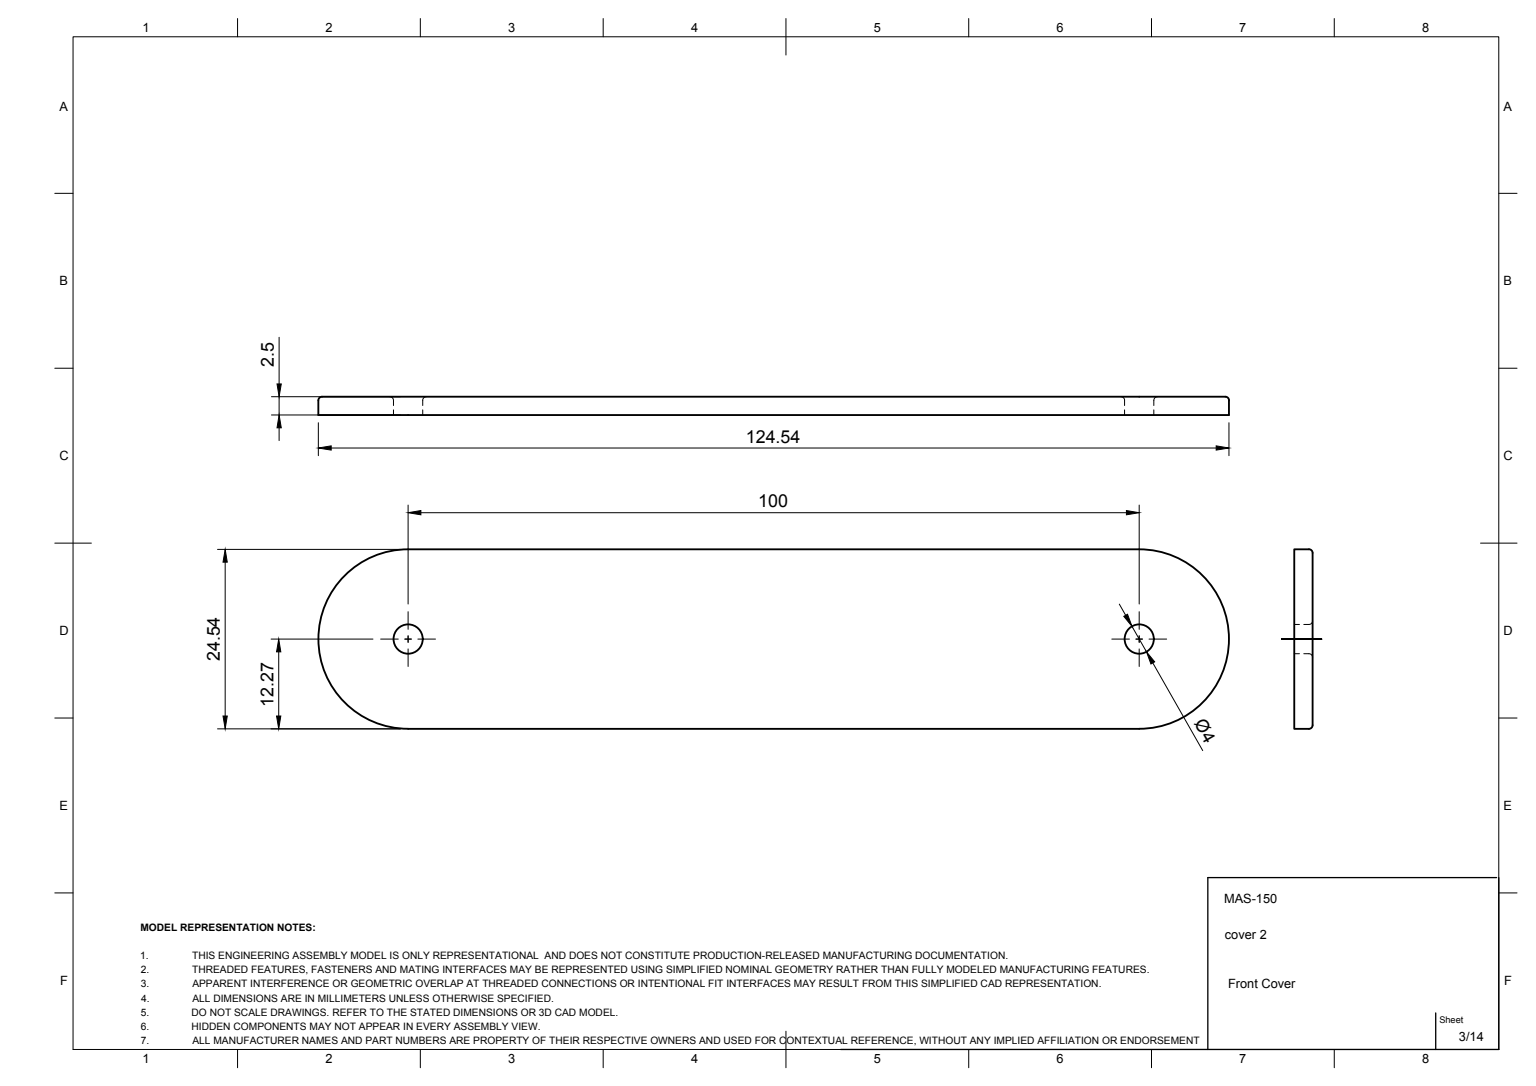
ISO-10303-21;
HEADER;
/* Generated by software containing ST-Developer
 * from STEP Tools, Inc. (www.steptools.com) 
 */

FILE_DESCRIPTION(
/* description */ ('STEP AP203'),
/* implementation_level */ '2;1');

FILE_NAME(
/* name */ 'Front Cover.step',
/* time_stamp */ '2026-11-08T21:40:52-08:00',
/* author */ (''),
/* organization */ (''),
/* preprocessor_version */ 'ST-DEVELOPER v20.2',
/* originating_system */ 'Autodesk Translation Framework v15.17.0.0',
/* authorisation */ '');

FILE_SCHEMA (('AUTOMOTIVE_DESIGN { 1 0 10303 214 3 1 1 }'));
ENDSEC;

DATA;
#10=MECHANICAL_DESIGN_GEOMETRIC_PRESENTATION_REPRESENTATION('',(#183),#12137);
#161=SHAPE_REPRESENTATION_RELATIONSHIP('SRR','None',#12184,#172);
#172=ADVANCED_BREP_SHAPE_REPRESENTATION('',(#194),#12125);
#183=STYLED_ITEM('',(#12253),#194);
#194=MANIFOLD_SOLID_BREP('Body1',#1828);
#205=FACE_BOUND('',#605,.T.);
#206=FACE_BOUND('',#606,.T.);
#207=FACE_BOUND('',#608,.T.);
#208=FACE_BOUND('',#609,.T.);
#232=PLANE('',#1977);
#233=PLANE('',#1980);
#234=PLANE('',#1985);
#235=PLANE('',#1988);
#276=LINE('',#2672,#370);
#277=LINE('',#2676,#371);
#278=LINE('',#2683,#372);
#279=LINE('',#2686,#373);
#280=LINE('',#2692,#374);
#281=LINE('',#2695,#375);
#282=LINE('',#2698,#376);
#283=LINE('',#2701,#377);
#284=LINE('',#2704,#378);
#285=LINE('',#2705,#379);
#286=LINE('',#2708,#380);
#287=LINE('',#2711,#381);
#370=VECTOR('',#2186,2.);
#371=VECTOR('',#2191,2.);
#372=VECTOR('',#2198,1000.);
#373=VECTOR('',#2201,1000.);
#374=VECTOR('',#2206,1000.);
#375=VECTOR('',#2209,1000.);
#376=VECTOR('',#2212,1000.);
#377=VECTOR('',#2215,1000.);
#378=VECTOR('',#2218,1000.);
#379=VECTOR('',#2219,1000.);
#380=VECTOR('',#2222,1000.);
#381=VECTOR('',#2227,1000.);
#464=CYLINDRICAL_SURFACE('',#1973,2.);
#465=CYLINDRICAL_SURFACE('',#1975,2.);
#466=CYLINDRICAL_SURFACE('',#1983,12.2723008899906);
#467=CYLINDRICAL_SURFACE('',#1986,12.2723008899906);
#468=CYLINDRICAL_SURFACE('',#1989,0.5);
#469=CYLINDRICAL_SURFACE('',#1996,0.5);
#490=FACE_OUTER_BOUND('',#600,.T.);
#491=FACE_OUTER_BOUND('',#601,.T.);
#492=FACE_OUTER_BOUND('',#602,.T.);
#493=FACE_OUTER_BOUND('',#603,.T.);
#494=FACE_OUTER_BOUND('',#604,.T.);
#495=FACE_OUTER_BOUND('',#607,.T.);
#496=FACE_OUTER_BOUND('',#610,.T.);
#497=FACE_OUTER_BOUND('',#611,.T.);
#498=FACE_OUTER_BOUND('',#612,.T.);
#499=FACE_OUTER_BOUND('',#613,.T.);
#500=FACE_OUTER_BOUND('',#614,.T.);
#501=FACE_OUTER_BOUND('',#615,.T.);
#502=FACE_OUTER_BOUND('',#616,.T.);
#503=FACE_OUTER_BOUND('',#617,.T.);
#600=EDGE_LOOP('',(#1223,#1224,#1225,#1226,#1227));
#601=EDGE_LOOP('',(#1228,#1229,#1230,#1231,#1232));
#602=EDGE_LOOP('',(#1233,#1234,#1235,#1236,#1237));
#603=EDGE_LOOP('',(#1238,#1239,#1240,#1241,#1242));
#604=EDGE_LOOP('',(#1243,#1244,#1245,#1246));
#605=EDGE_LOOP('',(#1247));
#606=EDGE_LOOP('',(#1248));
#607=EDGE_LOOP('',(#1249,#1250,#1251,#1252));
#608=EDGE_LOOP('',(#1253));
#609=EDGE_LOOP('',(#1254));
#610=EDGE_LOOP('',(#1255,#1256,#1257,#1258));
#611=EDGE_LOOP('',(#1259,#1260,#1261,#1262));
#612=EDGE_LOOP('',(#1263,#1264,#1265,#1266));
#613=EDGE_LOOP('',(#1267,#1268,#1269,#1270));
#614=EDGE_LOOP('',(#1271,#1272,#1273,#1274));
#615=EDGE_LOOP('',(#1275,#1276,#1277,#1278));
#616=EDGE_LOOP('',(#1279,#1280,#1281,#1282));
#617=EDGE_LOOP('',(#1283,#1284,#1285,#1286));
#737=CIRCLE('',#1964,2.);
#738=CIRCLE('',#1965,2.);
#739=CIRCLE('',#1966,0.5);
#740=CIRCLE('',#1967,2.5);
#741=CIRCLE('',#1969,2.);
#742=CIRCLE('',#1970,2.);
#743=CIRCLE('',#1971,0.5);
#744=CIRCLE('',#1972,2.5);
#745=CIRCLE('',#1974,2.);
#746=CIRCLE('',#1976,2.);
#747=CIRCLE('',#1978,11.7723008899906);
#748=CIRCLE('',#1979,11.7723008899906);
#749=CIRCLE('',#1981,12.2723008899906);
#750=CIRCLE('',#1982,12.2723008899906);
#751=CIRCLE('',#1984,12.2723008899906);
#752=CIRCLE('',#1987,12.2723008899906);
#753=CIRCLE('',#1990,0.5);
#754=CIRCLE('',#1991,0.5);
#755=CIRCLE('',#1993,0.5);
#756=CIRCLE('',#1995,0.5);
#824=VERTEX_POINT('',#2655);
#825=VERTEX_POINT('',#2656);
#826=VERTEX_POINT('',#2659);
#827=VERTEX_POINT('',#2663);
#828=VERTEX_POINT('',#2664);
#829=VERTEX_POINT('',#2667);
#830=VERTEX_POINT('',#2671);
#831=VERTEX_POINT('',#2675);
#832=VERTEX_POINT('',#2679);
#833=VERTEX_POINT('',#2680);
#834=VERTEX_POINT('',#2682);
#835=VERTEX_POINT('',#2684);
#836=VERTEX_POINT('',#2688);
#837=VERTEX_POINT('',#2689);
#838=VERTEX_POINT('',#2691);
#839=VERTEX_POINT('',#2693);
#840=VERTEX_POINT('',#2697);
#841=VERTEX_POINT('',#2699);
#842=VERTEX_POINT('',#2703);
#843=VERTEX_POINT('',#2707);
#981=EDGE_CURVE('',#824,#825,#737,.T.);
#982=EDGE_CURVE('',#825,#824,#738,.T.);
#983=EDGE_CURVE('',#825,#826,#739,.T.);
#984=EDGE_CURVE('',#826,#826,#740,.T.);
#985=EDGE_CURVE('',#827,#828,#741,.T.);
#986=EDGE_CURVE('',#828,#827,#742,.T.);
#987=EDGE_CURVE('',#828,#829,#743,.T.);
#988=EDGE_CURVE('',#829,#829,#744,.T.);
#989=EDGE_CURVE('',#827,#830,#276,.T.);
#990=EDGE_CURVE('',#830,#830,#745,.T.);
#991=EDGE_CURVE('',#824,#831,#277,.T.);
#992=EDGE_CURVE('',#831,#831,#746,.T.);
#993=EDGE_CURVE('',#832,#833,#747,.T.);
#994=EDGE_CURVE('',#833,#834,#278,.T.);
#995=EDGE_CURVE('',#834,#835,#748,.T.);
#996=EDGE_CURVE('',#835,#832,#279,.T.);
#997=EDGE_CURVE('',#836,#837,#749,.T.);
#998=EDGE_CURVE('',#838,#836,#280,.T.);
#999=EDGE_CURVE('',#839,#838,#750,.T.);
#1000=EDGE_CURVE('',#837,#839,#281,.T.);
#1001=EDGE_CURVE('',#840,#837,#282,.T.);
#1002=EDGE_CURVE('',#840,#841,#751,.T.);
#1003=EDGE_CURVE('',#841,#836,#283,.T.);
#1004=EDGE_CURVE('',#842,#839,#284,.T.);
#1005=EDGE_CURVE('',#842,#840,#285,.T.);
#1006=EDGE_CURVE('',#843,#838,#286,.T.);
#1007=EDGE_CURVE('',#843,#842,#752,.T.);
#1008=EDGE_CURVE('',#841,#843,#287,.T.);
#1009=EDGE_CURVE('',#840,#835,#753,.T.);
#1010=EDGE_CURVE('',#832,#842,#754,.T.);
#1011=EDGE_CURVE('',#833,#843,#755,.T.);
#1012=EDGE_CURVE('',#841,#834,#756,.T.);
#1223=ORIENTED_EDGE('',*,*,#981,.F.);
#1224=ORIENTED_EDGE('',*,*,#982,.F.);
#1225=ORIENTED_EDGE('',*,*,#983,.T.);
#1226=ORIENTED_EDGE('',*,*,#984,.F.);
#1227=ORIENTED_EDGE('',*,*,#983,.F.);
#1228=ORIENTED_EDGE('',*,*,#985,.F.);
#1229=ORIENTED_EDGE('',*,*,#986,.F.);
#1230=ORIENTED_EDGE('',*,*,#987,.T.);
#1231=ORIENTED_EDGE('',*,*,#988,.F.);
#1232=ORIENTED_EDGE('',*,*,#987,.F.);
#1233=ORIENTED_EDGE('',*,*,#985,.T.);
#1234=ORIENTED_EDGE('',*,*,#986,.T.);
#1235=ORIENTED_EDGE('',*,*,#989,.T.);
#1236=ORIENTED_EDGE('',*,*,#990,.F.);
#1237=ORIENTED_EDGE('',*,*,#989,.F.);
#1238=ORIENTED_EDGE('',*,*,#981,.T.);
#1239=ORIENTED_EDGE('',*,*,#982,.T.);
#1240=ORIENTED_EDGE('',*,*,#991,.T.);
#1241=ORIENTED_EDGE('',*,*,#992,.F.);
#1242=ORIENTED_EDGE('',*,*,#991,.F.);
#1243=ORIENTED_EDGE('',*,*,#993,.T.);
#1244=ORIENTED_EDGE('',*,*,#994,.T.);
#1245=ORIENTED_EDGE('',*,*,#995,.T.);
#1246=ORIENTED_EDGE('',*,*,#996,.T.);
#1247=ORIENTED_EDGE('',*,*,#984,.T.);
#1248=ORIENTED_EDGE('',*,*,#988,.T.);
#1249=ORIENTED_EDGE('',*,*,#997,.F.);
#1250=ORIENTED_EDGE('',*,*,#998,.F.);
#1251=ORIENTED_EDGE('',*,*,#999,.F.);
#1252=ORIENTED_EDGE('',*,*,#1000,.F.);
#1253=ORIENTED_EDGE('',*,*,#992,.T.);
#1254=ORIENTED_EDGE('',*,*,#990,.T.);
#1255=ORIENTED_EDGE('',*,*,#1001,.F.);
#1256=ORIENTED_EDGE('',*,*,#1002,.T.);
#1257=ORIENTED_EDGE('',*,*,#1003,.T.);
#1258=ORIENTED_EDGE('',*,*,#997,.T.);
#1259=ORIENTED_EDGE('',*,*,#1004,.F.);
#1260=ORIENTED_EDGE('',*,*,#1005,.T.);
#1261=ORIENTED_EDGE('',*,*,#1001,.T.);
#1262=ORIENTED_EDGE('',*,*,#1000,.T.);
#1263=ORIENTED_EDGE('',*,*,#1006,.F.);
#1264=ORIENTED_EDGE('',*,*,#1007,.T.);
#1265=ORIENTED_EDGE('',*,*,#1004,.T.);
#1266=ORIENTED_EDGE('',*,*,#999,.T.);
#1267=ORIENTED_EDGE('',*,*,#1003,.F.);
#1268=ORIENTED_EDGE('',*,*,#1008,.T.);
#1269=ORIENTED_EDGE('',*,*,#1006,.T.);
#1270=ORIENTED_EDGE('',*,*,#998,.T.);
#1271=ORIENTED_EDGE('',*,*,#1009,.F.);
#1272=ORIENTED_EDGE('',*,*,#1005,.F.);
#1273=ORIENTED_EDGE('',*,*,#1010,.F.);
#1274=ORIENTED_EDGE('',*,*,#996,.F.);
#1275=ORIENTED_EDGE('',*,*,#1010,.T.);
#1276=ORIENTED_EDGE('',*,*,#1007,.F.);
#1277=ORIENTED_EDGE('',*,*,#1011,.F.);
#1278=ORIENTED_EDGE('',*,*,#993,.F.);
#1279=ORIENTED_EDGE('',*,*,#1009,.T.);
#1280=ORIENTED_EDGE('',*,*,#995,.F.);
#1281=ORIENTED_EDGE('',*,*,#1012,.F.);
#1282=ORIENTED_EDGE('',*,*,#1002,.F.);
#1283=ORIENTED_EDGE('',*,*,#1011,.T.);
#1284=ORIENTED_EDGE('',*,*,#1008,.F.);
#1285=ORIENTED_EDGE('',*,*,#1012,.T.);
#1286=ORIENTED_EDGE('',*,*,#994,.F.);
#1707=TOROIDAL_SURFACE('',#1963,2.5,0.5);
#1708=TOROIDAL_SURFACE('',#1968,2.5,0.5);
#1709=TOROIDAL_SURFACE('',#1992,11.7723008899906,0.5);
#1710=TOROIDAL_SURFACE('',#1994,11.7723008899906,0.5);
#1718=ADVANCED_FACE('',(#490),#1707,.T.);
#1719=ADVANCED_FACE('',(#491),#1708,.T.);
#1720=ADVANCED_FACE('',(#492),#464,.F.);
#1721=ADVANCED_FACE('',(#493),#465,.F.);
#1722=ADVANCED_FACE('',(#494,#205,#206),#232,.T.);
#1723=ADVANCED_FACE('',(#495,#207,#208),#233,.F.);
#1724=ADVANCED_FACE('',(#496),#466,.T.);
#1725=ADVANCED_FACE('',(#497),#234,.F.);
#1726=ADVANCED_FACE('',(#498),#467,.T.);
#1727=ADVANCED_FACE('',(#499),#235,.F.);
#1728=ADVANCED_FACE('',(#500),#468,.T.);
#1729=ADVANCED_FACE('',(#501),#1709,.T.);
#1730=ADVANCED_FACE('',(#502),#1710,.T.);
#1731=ADVANCED_FACE('',(#503),#469,.T.);
#1828=CLOSED_SHELL('',(#1718,#1719,#1720,#1721,#1722,#1723,#1724,#1725,
#1726,#1727,#1728,#1729,#1730,#1731));
#1962=AXIS2_PLACEMENT_3D('',#2653,#2162,#2163);
#1963=AXIS2_PLACEMENT_3D('',#2654,#2164,#2165);
#1964=AXIS2_PLACEMENT_3D('',#2657,#2166,#2167);
#1965=AXIS2_PLACEMENT_3D('',#2658,#2168,#2169);
#1966=AXIS2_PLACEMENT_3D('',#2660,#2170,#2171);
#1967=AXIS2_PLACEMENT_3D('',#2661,#2172,#2173);
#1968=AXIS2_PLACEMENT_3D('',#2662,#2174,#2175);
#1969=AXIS2_PLACEMENT_3D('',#2665,#2176,#2177);
#1970=AXIS2_PLACEMENT_3D('',#2666,#2178,#2179);
#1971=AXIS2_PLACEMENT_3D('',#2668,#2180,#2181);
#1972=AXIS2_PLACEMENT_3D('',#2669,#2182,#2183);
#1973=AXIS2_PLACEMENT_3D('',#2670,#2184,#2185);
#1974=AXIS2_PLACEMENT_3D('',#2673,#2187,#2188);
#1975=AXIS2_PLACEMENT_3D('',#2674,#2189,#2190);
#1976=AXIS2_PLACEMENT_3D('',#2677,#2192,#2193);
#1977=AXIS2_PLACEMENT_3D('',#2678,#2194,#2195);
#1978=AXIS2_PLACEMENT_3D('',#2681,#2196,#2197);
#1979=AXIS2_PLACEMENT_3D('',#2685,#2199,#2200);
#1980=AXIS2_PLACEMENT_3D('',#2687,#2202,#2203);
#1981=AXIS2_PLACEMENT_3D('',#2690,#2204,#2205);
#1982=AXIS2_PLACEMENT_3D('',#2694,#2207,#2208);
#1983=AXIS2_PLACEMENT_3D('',#2696,#2210,#2211);
#1984=AXIS2_PLACEMENT_3D('',#2700,#2213,#2214);
#1985=AXIS2_PLACEMENT_3D('',#2702,#2216,#2217);
#1986=AXIS2_PLACEMENT_3D('',#2706,#2220,#2221);
#1987=AXIS2_PLACEMENT_3D('',#2709,#2223,#2224);
#1988=AXIS2_PLACEMENT_3D('',#2710,#2225,#2226);
#1989=AXIS2_PLACEMENT_3D('',#2712,#2228,#2229);
#1990=AXIS2_PLACEMENT_3D('',#2713,#2230,#2231);
#1991=AXIS2_PLACEMENT_3D('',#2714,#2232,#2233);
#1992=AXIS2_PLACEMENT_3D('',#2715,#2234,#2235);
#1993=AXIS2_PLACEMENT_3D('',#2716,#2236,#2237);
#1994=AXIS2_PLACEMENT_3D('',#2717,#2238,#2239);
#1995=AXIS2_PLACEMENT_3D('',#2718,#2240,#2241);
#1996=AXIS2_PLACEMENT_3D('',#2719,#2242,#2243);
#2162=DIRECTION('axis',(0.,0.,1.));
#2163=DIRECTION('refdir',(1.,0.,0.));
#2164=DIRECTION('center_axis',(0.,1.,0.));
#2165=DIRECTION('ref_axis',(0.,0.,1.));
#2166=DIRECTION('center_axis',(0.,1.,0.));
#2167=DIRECTION('ref_axis',(0.,0.,1.));
#2168=DIRECTION('center_axis',(0.,1.,0.));
#2169=DIRECTION('ref_axis',(0.,0.,1.));
#2170=DIRECTION('center_axis',(-1.,0.,0.));
#2171=DIRECTION('ref_axis',(0.,0.,-1.));
#2172=DIRECTION('center_axis',(0.,-1.,0.));
#2173=DIRECTION('ref_axis',(0.,0.,1.));
#2174=DIRECTION('center_axis',(0.,1.,0.));
#2175=DIRECTION('ref_axis',(0.,0.,1.));
#2176=DIRECTION('center_axis',(0.,1.,0.));
#2177=DIRECTION('ref_axis',(0.,0.,1.));
#2178=DIRECTION('center_axis',(0.,1.,0.));
#2179=DIRECTION('ref_axis',(0.,0.,1.));
#2180=DIRECTION('center_axis',(-1.,0.,0.));
#2181=DIRECTION('ref_axis',(0.,0.,-1.));
#2182=DIRECTION('center_axis',(0.,-1.,0.));
#2183=DIRECTION('ref_axis',(0.,0.,1.));
#2184=DIRECTION('center_axis',(0.,-1.,0.));
#2185=DIRECTION('ref_axis',(0.,0.,-1.));
#2186=DIRECTION('',(0.,-1.,0.));
#2187=DIRECTION('center_axis',(0.,1.,0.));
#2188=DIRECTION('ref_axis',(0.,0.,1.));
#2189=DIRECTION('center_axis',(0.,-1.,0.));
#2190=DIRECTION('ref_axis',(0.,0.,-1.));
#2191=DIRECTION('',(0.,-1.,0.));
#2192=DIRECTION('center_axis',(0.,1.,0.));
#2193=DIRECTION('ref_axis',(0.,0.,1.));
#2194=DIRECTION('center_axis',(0.,1.,0.));
#2195=DIRECTION('ref_axis',(0.,0.,1.));
#2196=DIRECTION('center_axis',(0.,1.,0.));
#2197=DIRECTION('ref_axis',(0.,0.,1.));
#2198=DIRECTION('',(1.,0.,-7.77156117237611E-15));
#2199=DIRECTION('center_axis',(0.,1.,0.));
#2200=DIRECTION('ref_axis',(0.,0.,1.));
#2201=DIRECTION('',(-1.,0.,7.77156117237609E-15));
#2202=DIRECTION('center_axis',(0.,1.,0.));
#2203=DIRECTION('ref_axis',(0.,0.,1.));
#2204=DIRECTION('center_axis',(0.,1.,0.));
#2205=DIRECTION('ref_axis',(0.,0.,1.));
#2206=DIRECTION('',(1.,0.,-7.77156117237611E-15));
#2207=DIRECTION('center_axis',(0.,1.,0.));
#2208=DIRECTION('ref_axis',(0.,0.,1.));
#2209=DIRECTION('',(-1.,0.,7.77156117237609E-15));
#2210=DIRECTION('center_axis',(0.,-1.,0.));
#2211=DIRECTION('ref_axis',(0.,0.,-1.));
#2212=DIRECTION('',(0.,-1.,0.));
#2213=DIRECTION('center_axis',(0.,-1.,0.));
#2214=DIRECTION('ref_axis',(0.,0.,1.));
#2215=DIRECTION('',(0.,-1.,0.));
#2216=DIRECTION('center_axis',(7.77156117237609E-15,0.,1.));
#2217=DIRECTION('ref_axis',(1.,0.,-7.77156117237609E-15));
#2218=DIRECTION('',(0.,-1.,0.));
#2219=DIRECTION('',(1.,0.,-7.77156117237609E-15));
#2220=DIRECTION('center_axis',(0.,-1.,0.));
#2221=DIRECTION('ref_axis',(0.,0.,-1.));
#2222=DIRECTION('',(0.,-1.,0.));
#2223=DIRECTION('center_axis',(0.,-1.,0.));
#2224=DIRECTION('ref_axis',(0.,0.,1.));
#2225=DIRECTION('center_axis',(-7.77156117237611E-15,0.,-1.));
#2226=DIRECTION('ref_axis',(-1.,0.,7.77156117237611E-15));
#2227=DIRECTION('',(-1.,0.,7.77156117237611E-15));
#2228=DIRECTION('center_axis',(1.,0.,-7.77156117237609E-15));
#2229=DIRECTION('ref_axis',(-7.77156117237609E-15,0.,-1.));
#2230=DIRECTION('center_axis',(1.,0.,-6.93889390390722E-15));
#2231=DIRECTION('ref_axis',(-6.93889390390722E-15,0.,-1.));
#2232=DIRECTION('center_axis',(-1.,0.,0.));
#2233=DIRECTION('ref_axis',(0.,0.,1.));
#2234=DIRECTION('center_axis',(0.,1.,0.));
#2235=DIRECTION('ref_axis',(0.,0.,1.));
#2236=DIRECTION('center_axis',(1.,0.,0.));
#2237=DIRECTION('ref_axis',(0.,0.,-1.));
#2238=DIRECTION('center_axis',(0.,1.,0.));
#2239=DIRECTION('ref_axis',(0.,0.,1.));
#2240=DIRECTION('center_axis',(-1.,-6.93889390390723E-15,0.));
#2241=DIRECTION('ref_axis',(6.93889390390723E-15,-1.,0.));
#2242=DIRECTION('center_axis',(-1.,0.,7.77156117237611E-15));
#2243=DIRECTION('ref_axis',(7.77156117237611E-15,0.,1.));
#2653=CARTESIAN_POINT('',(0.,0.,0.));
#2654=CARTESIAN_POINT('Origin',(-83.4892602927113,2.,28.6344795489034));
#2655=CARTESIAN_POINT('',(-83.4892602927113,2.,30.6344795489034));
#2656=CARTESIAN_POINT('',(-83.4892602927113,2.,26.6344795489034));
#2657=CARTESIAN_POINT('Origin',(-83.4892602927113,2.,28.6344795489034));
#2658=CARTESIAN_POINT('Origin',(-83.4892602927113,2.,28.6344795489034));
#2659=CARTESIAN_POINT('',(-83.4892602927113,2.5,26.1344795489034));
#2660=CARTESIAN_POINT('Origin',(-83.4892602927113,2.,26.1344795489034));
#2661=CARTESIAN_POINT('Origin',(-83.4892602927113,2.5,28.6344795489034));
#2662=CARTESIAN_POINT('Origin',(16.5107397072887,2.,28.6344795489026));
#2663=CARTESIAN_POINT('',(16.5107397072887,2.,30.6344795489026));
#2664=CARTESIAN_POINT('',(16.5107397072887,2.,26.6344795489026));
#2665=CARTESIAN_POINT('Origin',(16.5107397072887,2.,28.6344795489026));
#2666=CARTESIAN_POINT('Origin',(16.5107397072887,2.,28.6344795489026));
#2667=CARTESIAN_POINT('',(16.5107397072887,2.5,26.1344795489026));
#2668=CARTESIAN_POINT('Origin',(16.5107397072887,2.,26.1344795489026));
#2669=CARTESIAN_POINT('Origin',(16.5107397072887,2.5,28.6344795489026));
#2670=CARTESIAN_POINT('Origin',(16.5107397072887,2.5,28.6344795489026));
#2671=CARTESIAN_POINT('',(16.5107397072887,0.,30.6344795489026));
#2672=CARTESIAN_POINT('',(16.5107397072887,2.5,30.6344795489026));
#2673=CARTESIAN_POINT('Origin',(16.5107397072887,0.,28.6344795489026));
#2674=CARTESIAN_POINT('Origin',(-83.4892602927113,2.5,28.6344795489034));
#2675=CARTESIAN_POINT('',(-83.4892602927113,0.,30.6344795489034));
#2676=CARTESIAN_POINT('',(-83.4892602927113,2.5,30.6344795489034));
#2677=CARTESIAN_POINT('Origin',(-83.4892602927113,0.,28.6344795489034));
#2678=CARTESIAN_POINT('Origin',(16.5107397072887,2.5,28.6344795489026));
#2679=CARTESIAN_POINT('',(-83.4892602927114,2.5,16.8621786589128));
#2680=CARTESIAN_POINT('',(-83.4892602927112,2.5,40.4067804388939));
#2681=CARTESIAN_POINT('Origin',(-83.4892602927113,2.5,28.6344795489034));
#2682=CARTESIAN_POINT('',(16.5107397072887,2.5,40.4067804388932));
#2683=CARTESIAN_POINT('',(16.5107397072887,2.5,40.4067804388932));
#2684=CARTESIAN_POINT('',(16.5107397072887,2.5,16.862178658912));
#2685=CARTESIAN_POINT('Origin',(16.5107397072887,2.5,28.6344795489026));
#2686=CARTESIAN_POINT('',(-83.4892602927114,2.5,16.8621786589128));
#2687=CARTESIAN_POINT('Origin',(16.5107397072887,0.,28.6344795489026));
#2688=CARTESIAN_POINT('',(16.5107397072887,0.,40.9067804388932));
#2689=CARTESIAN_POINT('',(16.5107397072887,0.,16.362178658912));
#2690=CARTESIAN_POINT('Origin',(16.5107397072887,0.,28.6344795489026));
#2691=CARTESIAN_POINT('',(-83.4892602927112,0.,40.9067804388939));
#2692=CARTESIAN_POINT('',(16.5107397072887,0.,40.9067804388932));
#2693=CARTESIAN_POINT('',(-83.4892602927114,0.,16.3621786589128));
#2694=CARTESIAN_POINT('Origin',(-83.4892602927113,0.,28.6344795489034));
#2695=CARTESIAN_POINT('',(16.5107397072887,0.,16.362178658912));
#2696=CARTESIAN_POINT('Origin',(16.5107397072887,2.5,28.6344795489026));
#2697=CARTESIAN_POINT('',(16.5107397072887,2.,16.362178658912));
#2698=CARTESIAN_POINT('',(16.5107397072887,2.5,16.362178658912));
#2699=CARTESIAN_POINT('',(16.5107397072887,2.,40.9067804388932));
#2700=CARTESIAN_POINT('Origin',(16.5107397072887,2.,28.6344795489026));
#2701=CARTESIAN_POINT('',(16.5107397072887,2.5,40.9067804388932));
#2702=CARTESIAN_POINT('Origin',(16.5107397072887,2.5,16.362178658912));
#2703=CARTESIAN_POINT('',(-83.4892602927114,2.,16.3621786589128));
#2704=CARTESIAN_POINT('',(-83.4892602927114,2.5,16.3621786589128));
#2705=CARTESIAN_POINT('',(16.5107397072887,2.,16.362178658912));
#2706=CARTESIAN_POINT('Origin',(-83.4892602927113,2.5,28.6344795489034));
#2707=CARTESIAN_POINT('',(-83.4892602927112,2.,40.9067804388939));
#2708=CARTESIAN_POINT('',(-83.4892602927112,2.5,40.9067804388939));
#2709=CARTESIAN_POINT('Origin',(-83.4892602927113,2.,28.6344795489034));
#2710=CARTESIAN_POINT('Origin',(16.5107397072887,2.5,40.9067804388932));
#2711=CARTESIAN_POINT('',(-83.4892602927112,2.,40.9067804388939));
#2712=CARTESIAN_POINT('Origin',(16.5107397072886,2.,16.862178658912));
#2713=CARTESIAN_POINT('Origin',(16.5107397072887,2.,16.862178658912));
#2714=CARTESIAN_POINT('Origin',(-83.4892602927114,2.,16.8621786589128));
#2715=CARTESIAN_POINT('Origin',(-83.4892602927113,2.,28.6344795489034));
#2716=CARTESIAN_POINT('Origin',(-83.4892602927112,2.,40.4067804388939));
#2717=CARTESIAN_POINT('Origin',(16.5107397072887,2.,28.6344795489026));
#2718=CARTESIAN_POINT('Origin',(16.5107397072887,2.,40.4067804388932));
#2719=CARTESIAN_POINT('Origin',(16.5107397072888,2.,40.4067804388932));
#12111=UNCERTAINTY_MEASURE_WITH_UNIT(LENGTH_MEASURE(0.01),#12138,
'DISTANCE_ACCURACY_VALUE',
'Maximum model space distance between geometric entities at asserted c
onnectivities');
#12123=UNCERTAINTY_MEASURE_WITH_UNIT(LENGTH_MEASURE(0.01),#12138,
'DISTANCE_ACCURACY_VALUE',
'Maximum model space distance between geometric entities at asserted c
onnectivities');
#12125=(
GEOMETRIC_REPRESENTATION_CONTEXT(3)
GLOBAL_UNCERTAINTY_ASSIGNED_CONTEXT((#12111))
GLOBAL_UNIT_ASSIGNED_CONTEXT((#12138,#12140,#12141))
REPRESENTATION_CONTEXT('','3D')
);
#12137=(
GEOMETRIC_REPRESENTATION_CONTEXT(3)
GLOBAL_UNCERTAINTY_ASSIGNED_CONTEXT((#12123))
GLOBAL_UNIT_ASSIGNED_CONTEXT((#12138,#12140,#12141))
REPRESENTATION_CONTEXT('','3D')
);
#12138=(
LENGTH_UNIT()
NAMED_UNIT(*)
SI_UNIT(.MILLI.,.METRE.)
);
#12140=(
NAMED_UNIT(*)
PLANE_ANGLE_UNIT()
SI_UNIT($,.RADIAN.)
);
#12141=(
NAMED_UNIT(*)
SI_UNIT($,.STERADIAN.)
SOLID_ANGLE_UNIT()
);
#12143=SHAPE_DEFINITION_REPRESENTATION(#12156,#12184);
#12156=PRODUCT_DEFINITION_SHAPE('',$,#12198);
#12184=SHAPE_REPRESENTATION('',(#1962),#12125);
#12196=PRODUCT_DEFINITION_CONTEXT('part definition',#12237,'design');
#12198=PRODUCT_DEFINITION('cover 2','Front Cover',#12211,#12196);
#12211=PRODUCT_DEFINITION_FORMATION('',$,#12240);
#12237=APPLICATION_CONTEXT(
'Core Data for Automotive Mechanical Design Process');
#12238=PRODUCT_CONTEXT('part definition',#12237,'mechanical');
#12240=PRODUCT('cover 2','Front Cover',$,(#12238));
#12253=PRESENTATION_STYLE_ASSIGNMENT((#12255));
#12255=SURFACE_STYLE_USAGE(.BOTH.,#12257);
#12257=SURFACE_SIDE_STYLE('',(#12259));
#12259=SURFACE_STYLE_FILL_AREA(#12261);
#12261=FILL_AREA_STYLE('Opaque(23,69,131)',(#12263));
#12263=FILL_AREA_STYLE_COLOUR('Opaque(23,69,131)',#12265);
#12265=COLOUR_RGB('Opaque(23,69,131)',0.0901960784313725,0.270588235294118,
0.513725490196078);
ENDSEC;
END-ISO-10303-21;
